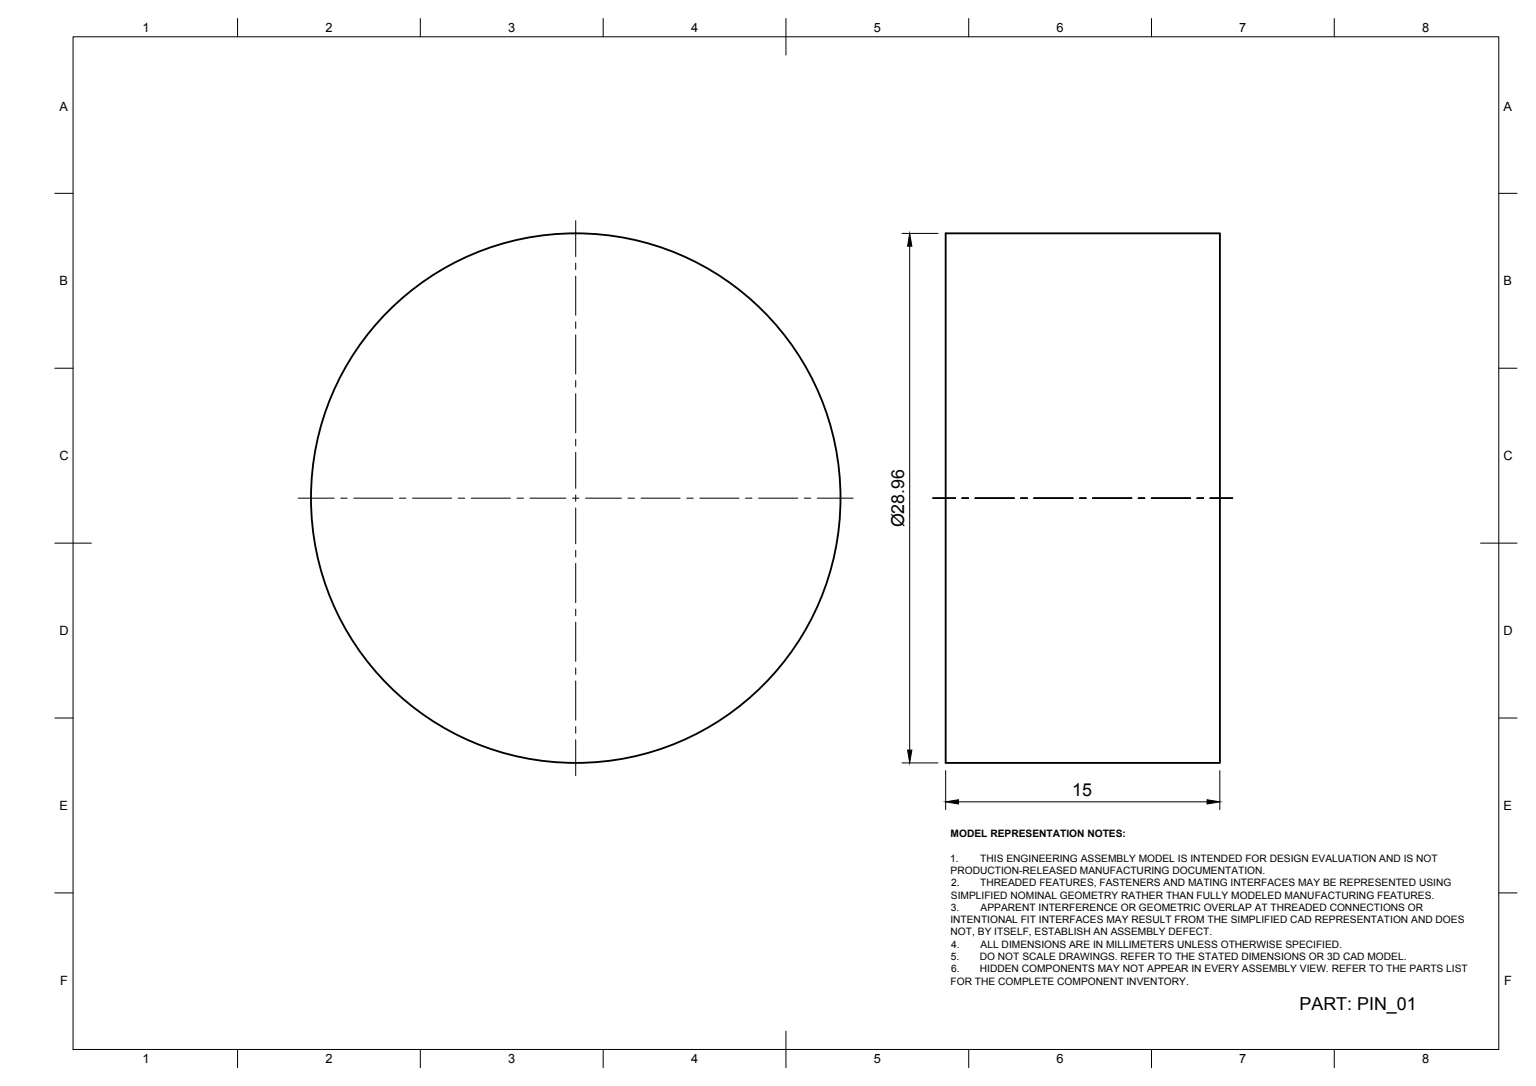
ISO-10303-21;
HEADER;
/* Generated by software containing ST-Developer
 * from STEP Tools, Inc. (www.steptools.com) 
 */

FILE_DESCRIPTION(
/* description */ (''),
/* implementation_level */ '2;1');

FILE_NAME(
/* name */ 'Pin_01.step',
/* time_stamp */ '2026-09-20T22:38:01+06:00',
/* author */ (''),
/* organization */ (''),
/* preprocessor_version */ 'ST-DEVELOPER v20.2',
/* originating_system */ 'Autodesk Translation Framework v15.15.0.0',
/* authorisation */ '');

FILE_SCHEMA (('AUTOMOTIVE_DESIGN { 1 0 10303 214 3 1 1 }'));
ENDSEC;

DATA;
#10=MECHANICAL_DESIGN_GEOMETRIC_PRESENTATION_REPRESENTATION('',(#91),#4079);
#75=SHAPE_REPRESENTATION_RELATIONSHIP('SRR','None',#4118,#83);
#83=ADVANCED_BREP_SHAPE_REPRESENTATION('',(#99),#4078);
#91=STYLED_ITEM('',(#4159),#99);
#99=MANIFOLD_SOLID_BREP('Pin_01',#1450);
#167=CIRCLE('',#1686,14.4819556358054);
#168=CIRCLE('',#1687,14.4819556358054);
#196=CYLINDRICAL_SURFACE('',#1685,14.4819556358054);
#278=FACE_OUTER_BOUND('',#368,.T.);
#279=FACE_OUTER_BOUND('',#369,.T.);
#280=FACE_OUTER_BOUND('',#370,.T.);
#368=EDGE_LOOP('',(#1303,#1304,#1305,#1306));
#369=EDGE_LOOP('',(#1307));
#370=EDGE_LOOP('',(#1308));
#483=LINE('',#4048,#596);
#596=VECTOR('',#2104,14.4819556358054);
#722=VERTEX_POINT('',#4045);
#723=VERTEX_POINT('',#4047);
#916=EDGE_CURVE('',#722,#722,#167,.T.);
#917=EDGE_CURVE('',#722,#723,#483,.T.);
#918=EDGE_CURVE('',#723,#723,#168,.T.);
#1303=ORIENTED_EDGE('',*,*,#916,.F.);
#1304=ORIENTED_EDGE('',*,*,#917,.T.);
#1305=ORIENTED_EDGE('',*,*,#918,.T.);
#1306=ORIENTED_EDGE('',*,*,#917,.F.);
#1307=ORIENTED_EDGE('',*,*,#916,.T.);
#1308=ORIENTED_EDGE('',*,*,#918,.F.);
#1357=PLANE('',#1688);
#1358=PLANE('',#1689);
#1440=ADVANCED_FACE('',(#278),#196,.T.);
#1441=ADVANCED_FACE('',(#279),#1357,.T.);
#1442=ADVANCED_FACE('',(#280),#1358,.F.);
#1450=CLOSED_SHELL('',(#1440,#1441,#1442));
#1684=AXIS2_PLACEMENT_3D('',#4043,#2098,#2099);
#1685=AXIS2_PLACEMENT_3D('',#4044,#2100,#2101);
#1686=AXIS2_PLACEMENT_3D('',#4046,#2102,#2103);
#1687=AXIS2_PLACEMENT_3D('',#4049,#2105,#2106);
#1688=AXIS2_PLACEMENT_3D('',#4050,#2107,#2108);
#1689=AXIS2_PLACEMENT_3D('',#4051,#2109,#2110);
#2098=DIRECTION('axis',(0.,0.,1.));
#2099=DIRECTION('refdir',(1.,0.,0.));
#2100=DIRECTION('center_axis',(0.,-1.,0.));
#2101=DIRECTION('ref_axis',(1.,0.,0.));
#2102=DIRECTION('center_axis',(0.,-1.,0.));
#2103=DIRECTION('ref_axis',(1.,0.,0.));
#2104=DIRECTION('',(0.,1.,0.));
#2105=DIRECTION('center_axis',(0.,-1.,0.));
#2106=DIRECTION('ref_axis',(1.,0.,0.));
#2107=DIRECTION('center_axis',(0.,-1.,0.));
#2108=DIRECTION('ref_axis',(1.,0.,0.));
#2109=DIRECTION('center_axis',(0.,-1.,0.));
#2110=DIRECTION('ref_axis',(1.,0.,0.));
#4043=CARTESIAN_POINT('',(0.,0.,0.));
#4044=CARTESIAN_POINT('Origin',(-0.00360820116592981,5.,47.167824608198));
#4045=CARTESIAN_POINT('',(-14.4855638369713,-10.,47.167824608198));
#4046=CARTESIAN_POINT('Origin',(-0.00360820116592981,-10.,47.167824608198));
#4047=CARTESIAN_POINT('',(-14.4855638369713,5.,47.167824608198));
#4048=CARTESIAN_POINT('',(-14.4855638369713,5.,47.167824608198));
#4049=CARTESIAN_POINT('Origin',(-0.00360820116592981,5.,47.167824608198));
#4050=CARTESIAN_POINT('Origin',(-0.00360820116592997,-10.,47.167824608198));
#4051=CARTESIAN_POINT('Origin',(-0.00360820116592997,5.,47.167824608198));
#4068=UNCERTAINTY_MEASURE_WITH_UNIT(LENGTH_MEASURE(0.01),#4080,
'DISTANCE_ACCURACY_VALUE',
'Maximum model space distance between geometric entities at asserted c
onnectivities');
#4069=UNCERTAINTY_MEASURE_WITH_UNIT(LENGTH_MEASURE(0.01),#4080,
'DISTANCE_ACCURACY_VALUE',
'Maximum model space distance between geometric entities at asserted c
onnectivities');
#4078=(
GEOMETRIC_REPRESENTATION_CONTEXT(3)
GLOBAL_UNCERTAINTY_ASSIGNED_CONTEXT((#4068))
GLOBAL_UNIT_ASSIGNED_CONTEXT((#4080,#4082,#4083))
REPRESENTATION_CONTEXT('','3D')
);
#4079=(
GEOMETRIC_REPRESENTATION_CONTEXT(3)
GLOBAL_UNCERTAINTY_ASSIGNED_CONTEXT((#4069))
GLOBAL_UNIT_ASSIGNED_CONTEXT((#4080,#4082,#4083))
REPRESENTATION_CONTEXT('','3D')
);
#4080=(
LENGTH_UNIT()
NAMED_UNIT(*)
SI_UNIT(.MILLI.,.METRE.)
);
#4082=(
NAMED_UNIT(*)
PLANE_ANGLE_UNIT()
SI_UNIT($,.RADIAN.)
);
#4083=(
NAMED_UNIT(*)
SI_UNIT($,.STERADIAN.)
SOLID_ANGLE_UNIT()
);
#4092=SHAPE_DEFINITION_REPRESENTATION(#4101,#4118);
#4101=PRODUCT_DEFINITION_SHAPE('',$,#4128);
#4118=SHAPE_REPRESENTATION('',(#1684),#4078);
#4119=PRODUCT_DEFINITION_CONTEXT('part definition',#4148,'design');
#4128=PRODUCT_DEFINITION('Pin_01','Pin_01',#4137,#4119);
#4137=PRODUCT_DEFINITION_FORMATION('',$,#4158);
#4148=APPLICATION_CONTEXT(
'Core Data for Automotive Mechanical Design Process');
#4149=PRODUCT_CONTEXT('part definition',#4148,'mechanical');
#4158=PRODUCT('Pin_01','Pin_01',$,(#4149));
#4159=PRESENTATION_STYLE_ASSIGNMENT((#4163));
#4163=SURFACE_STYLE_USAGE(.BOTH.,#4167);
#4167=SURFACE_SIDE_STYLE('',(#4171));
#4171=SURFACE_STYLE_FILL_AREA(#4175);
#4175=FILL_AREA_STYLE('Steel - Satin',(#4179));
#4179=FILL_AREA_STYLE_COLOUR('Steel - Satin',#4183);
#4183=COLOUR_RGB('Steel - Satin', 0.40784314, 0.44705882, 0.49803922);
ENDSEC;
END-ISO-10303-21;
